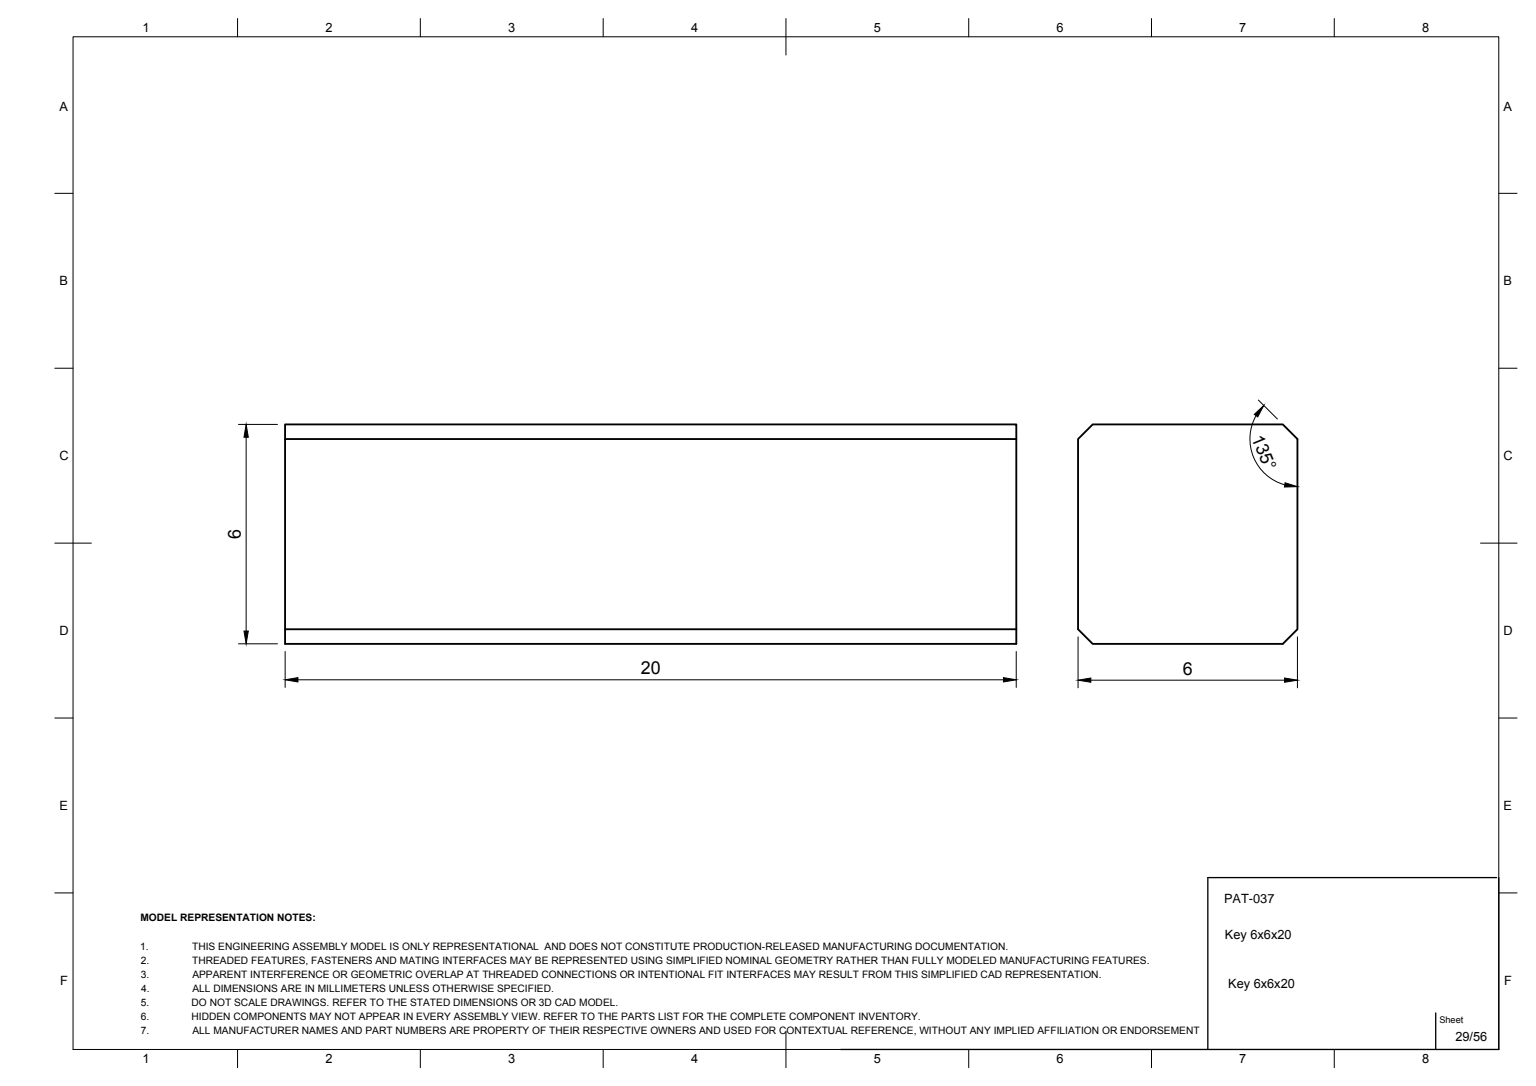
ISO-10303-21;
HEADER;
/* Generated by software containing ST-Developer
 * from STEP Tools, Inc. (www.steptools.com) 
 */

FILE_DESCRIPTION(
/* description */ ('Flywheel Crank-Slider'),
/* implementation_level */ '2;1');

FILE_NAME(
/* name */ 'Key 6x6x20.step',
/* time_stamp */ '2026-10-28T03:23:13-07:00',
/* author */ (''),
/* organization */ (''),
/* preprocessor_version */ 'ST-DEVELOPER v20.2',
/* originating_system */ 'Autodesk Translation Framework v15.17.0.0',
/* authorisation */ '');

FILE_SCHEMA (('AUTOMOTIVE_DESIGN { 1 0 10303 214 3 1 1 }'));
ENDSEC;

DATA;
#10=MECHANICAL_DESIGN_GEOMETRIC_PRESENTATION_REPRESENTATION('',(#699),#17322);
#594=SHAPE_REPRESENTATION_RELATIONSHIP('SRR','None',#17592,#646);
#646=ADVANCED_BREP_SHAPE_REPRESENTATION('',(#756),#17296);
#699=STYLED_ITEM('',(#17931),#756);
#756=MANIFOLD_SOLID_BREP('Body1',#9081);
#1211=PLANE('',#10312);
#1212=PLANE('',#10313);
#1213=PLANE('',#10314);
#1214=PLANE('',#10315);
#1215=PLANE('',#10316);
#1216=PLANE('',#10317);
#1217=PLANE('',#10318);
#1218=PLANE('',#10319);
#1219=PLANE('',#10320);
#1220=PLANE('',#10321);
#1656=FACE_OUTER_BOUND('',#2336,.T.);
#1657=FACE_OUTER_BOUND('',#2337,.T.);
#1658=FACE_OUTER_BOUND('',#2338,.T.);
#1659=FACE_OUTER_BOUND('',#2339,.T.);
#1660=FACE_OUTER_BOUND('',#2340,.T.);
#1661=FACE_OUTER_BOUND('',#2341,.T.);
#1662=FACE_OUTER_BOUND('',#2342,.T.);
#1663=FACE_OUTER_BOUND('',#2343,.T.);
#1664=FACE_OUTER_BOUND('',#2344,.T.);
#1665=FACE_OUTER_BOUND('',#2345,.T.);
#2336=EDGE_LOOP('',(#7516,#7517,#7518,#7519,#7520,#7521,#7522,#7523));
#2337=EDGE_LOOP('',(#7524,#7525,#7526,#7527));
#2338=EDGE_LOOP('',(#7528,#7529,#7530,#7531));
#2339=EDGE_LOOP('',(#7532,#7533,#7534,#7535));
#2340=EDGE_LOOP('',(#7536,#7537,#7538,#7539));
#2341=EDGE_LOOP('',(#7540,#7541,#7542,#7543,#7544,#7545,#7546,#7547));
#2342=EDGE_LOOP('',(#7548,#7549,#7550,#7551));
#2343=EDGE_LOOP('',(#7552,#7553,#7554,#7555));
#2344=EDGE_LOOP('',(#7556,#7557,#7558,#7559));
#2345=EDGE_LOOP('',(#7560,#7561,#7562,#7563));
#3023=LINE('',#15847,#3634);
#3024=LINE('',#15849,#3635);
#3025=LINE('',#15851,#3636);
#3026=LINE('',#15853,#3637);
#3027=LINE('',#15855,#3638);
#3028=LINE('',#15857,#3639);
#3029=LINE('',#15859,#3640);
#3030=LINE('',#15860,#3641);
#3031=LINE('',#15863,#3642);
#3032=LINE('',#15865,#3643);
#3033=LINE('',#15866,#3644);
#3034=LINE('',#15869,#3645);
#3035=LINE('',#15870,#3646);
#3036=LINE('',#15873,#3647);
#3037=LINE('',#15874,#3648);
#3038=LINE('',#15877,#3649);
#3039=LINE('',#15878,#3650);
#3040=LINE('',#15882,#3651);
#3041=LINE('',#15883,#3652);
#3042=LINE('',#15885,#3653);
#3043=LINE('',#15886,#3654);
#3044=LINE('',#15888,#3655);
#3045=LINE('',#15890,#3656);
#3046=LINE('',#15892,#3657);
#3634=VECTOR('',#12493,1.);
#3635=VECTOR('',#12494,1.);
#3636=VECTOR('',#12495,1.);
#3637=VECTOR('',#12496,1.);
#3638=VECTOR('',#12497,1.);
#3639=VECTOR('',#12498,1.);
#3640=VECTOR('',#12499,1.);
#3641=VECTOR('',#12500,1.);
#3642=VECTOR('',#12503,1.);
#3643=VECTOR('',#12504,1.);
#3644=VECTOR('',#12505,1.);
#3645=VECTOR('',#12508,1.);
#3646=VECTOR('',#12509,1.);
#3647=VECTOR('',#12512,1.);
#3648=VECTOR('',#12513,1.);
#3649=VECTOR('',#12516,1.);
#3650=VECTOR('',#12517,1.);
#3651=VECTOR('',#12520,1.);
#3652=VECTOR('',#12521,1.);
#3653=VECTOR('',#12522,1.);
#3654=VECTOR('',#12523,1.);
#3655=VECTOR('',#12526,1.);
#3656=VECTOR('',#12529,1.);
#3657=VECTOR('',#12532,1.);
#4739=VERTEX_POINT('',#15845);
#4740=VERTEX_POINT('',#15846);
#4741=VERTEX_POINT('',#15848);
#4742=VERTEX_POINT('',#15850);
#4743=VERTEX_POINT('',#15852);
#4744=VERTEX_POINT('',#15854);
#4745=VERTEX_POINT('',#15856);
#4746=VERTEX_POINT('',#15858);
#4747=VERTEX_POINT('',#15862);
#4748=VERTEX_POINT('',#15864);
#4749=VERTEX_POINT('',#15868);
#4750=VERTEX_POINT('',#15872);
#4751=VERTEX_POINT('',#15876);
#4752=VERTEX_POINT('',#15880);
#4753=VERTEX_POINT('',#15881);
#4754=VERTEX_POINT('',#15884);
#5715=EDGE_CURVE('',#4739,#4740,#3023,.T.);
#5716=EDGE_CURVE('',#4741,#4739,#3024,.T.);
#5717=EDGE_CURVE('',#4742,#4741,#3025,.T.);
#5718=EDGE_CURVE('',#4743,#4742,#3026,.T.);
#5719=EDGE_CURVE('',#4744,#4743,#3027,.T.);
#5720=EDGE_CURVE('',#4745,#4744,#3028,.T.);
#5721=EDGE_CURVE('',#4746,#4745,#3029,.T.);
#5722=EDGE_CURVE('',#4740,#4746,#3030,.T.);
#5723=EDGE_CURVE('',#4743,#4747,#3031,.T.);
#5724=EDGE_CURVE('',#4747,#4748,#3032,.T.);
#5725=EDGE_CURVE('',#4748,#4744,#3033,.T.);
#5726=EDGE_CURVE('',#4749,#4742,#3034,.T.);
#5727=EDGE_CURVE('',#4749,#4747,#3035,.T.);
#5728=EDGE_CURVE('',#4741,#4750,#3036,.T.);
#5729=EDGE_CURVE('',#4750,#4749,#3037,.T.);
#5730=EDGE_CURVE('',#4751,#4739,#3038,.T.);
#5731=EDGE_CURVE('',#4751,#4750,#3039,.T.);
#5732=EDGE_CURVE('',#4752,#4753,#3040,.T.);
#5733=EDGE_CURVE('',#4748,#4752,#3041,.T.);
#5734=EDGE_CURVE('',#4754,#4751,#3042,.T.);
#5735=EDGE_CURVE('',#4753,#4754,#3043,.T.);
#5736=EDGE_CURVE('',#4745,#4752,#3044,.T.);
#5737=EDGE_CURVE('',#4740,#4754,#3045,.T.);
#5738=EDGE_CURVE('',#4753,#4746,#3046,.T.);
#7516=ORIENTED_EDGE('',*,*,#5715,.F.);
#7517=ORIENTED_EDGE('',*,*,#5716,.F.);
#7518=ORIENTED_EDGE('',*,*,#5717,.F.);
#7519=ORIENTED_EDGE('',*,*,#5718,.F.);
#7520=ORIENTED_EDGE('',*,*,#5719,.F.);
#7521=ORIENTED_EDGE('',*,*,#5720,.F.);
#7522=ORIENTED_EDGE('',*,*,#5721,.F.);
#7523=ORIENTED_EDGE('',*,*,#5722,.F.);
#7524=ORIENTED_EDGE('',*,*,#5719,.T.);
#7525=ORIENTED_EDGE('',*,*,#5723,.T.);
#7526=ORIENTED_EDGE('',*,*,#5724,.T.);
#7527=ORIENTED_EDGE('',*,*,#5725,.T.);
#7528=ORIENTED_EDGE('',*,*,#5718,.T.);
#7529=ORIENTED_EDGE('',*,*,#5726,.F.);
#7530=ORIENTED_EDGE('',*,*,#5727,.T.);
#7531=ORIENTED_EDGE('',*,*,#5723,.F.);
#7532=ORIENTED_EDGE('',*,*,#5717,.T.);
#7533=ORIENTED_EDGE('',*,*,#5728,.T.);
#7534=ORIENTED_EDGE('',*,*,#5729,.T.);
#7535=ORIENTED_EDGE('',*,*,#5726,.T.);
#7536=ORIENTED_EDGE('',*,*,#5716,.T.);
#7537=ORIENTED_EDGE('',*,*,#5730,.F.);
#7538=ORIENTED_EDGE('',*,*,#5731,.T.);
#7539=ORIENTED_EDGE('',*,*,#5728,.F.);
#7540=ORIENTED_EDGE('',*,*,#5732,.F.);
#7541=ORIENTED_EDGE('',*,*,#5733,.F.);
#7542=ORIENTED_EDGE('',*,*,#5724,.F.);
#7543=ORIENTED_EDGE('',*,*,#5727,.F.);
#7544=ORIENTED_EDGE('',*,*,#5729,.F.);
#7545=ORIENTED_EDGE('',*,*,#5731,.F.);
#7546=ORIENTED_EDGE('',*,*,#5734,.F.);
#7547=ORIENTED_EDGE('',*,*,#5735,.F.);
#7548=ORIENTED_EDGE('',*,*,#5720,.T.);
#7549=ORIENTED_EDGE('',*,*,#5725,.F.);
#7550=ORIENTED_EDGE('',*,*,#5733,.T.);
#7551=ORIENTED_EDGE('',*,*,#5736,.F.);
#7552=ORIENTED_EDGE('',*,*,#5715,.T.);
#7553=ORIENTED_EDGE('',*,*,#5737,.T.);
#7554=ORIENTED_EDGE('',*,*,#5734,.T.);
#7555=ORIENTED_EDGE('',*,*,#5730,.T.);
#7556=ORIENTED_EDGE('',*,*,#5721,.T.);
#7557=ORIENTED_EDGE('',*,*,#5736,.T.);
#7558=ORIENTED_EDGE('',*,*,#5732,.T.);
#7559=ORIENTED_EDGE('',*,*,#5738,.T.);
#7560=ORIENTED_EDGE('',*,*,#5722,.T.);
#7561=ORIENTED_EDGE('',*,*,#5738,.F.);
#7562=ORIENTED_EDGE('',*,*,#5735,.T.);
#7563=ORIENTED_EDGE('',*,*,#5737,.F.);
#8847=ADVANCED_FACE('',(#1656),#1211,.F.);
#8848=ADVANCED_FACE('',(#1657),#1212,.T.);
#8849=ADVANCED_FACE('',(#1658),#1213,.T.);
#8850=ADVANCED_FACE('',(#1659),#1214,.T.);
#8851=ADVANCED_FACE('',(#1660),#1215,.T.);
#8852=ADVANCED_FACE('',(#1661),#1216,.T.);
#8853=ADVANCED_FACE('',(#1662),#1217,.F.);
#8854=ADVANCED_FACE('',(#1663),#1218,.T.);
#8855=ADVANCED_FACE('',(#1664),#1219,.T.);
#8856=ADVANCED_FACE('',(#1665),#1220,.T.);
#9081=CLOSED_SHELL('',(#8847,#8848,#8849,#8850,#8851,#8852,#8853,#8854,
#8855,#8856));
#10311=AXIS2_PLACEMENT_3D('',#15843,#12489,#12490);
#10312=AXIS2_PLACEMENT_3D('',#15844,#12491,#12492);
#10313=AXIS2_PLACEMENT_3D('',#15861,#12501,#12502);
#10314=AXIS2_PLACEMENT_3D('',#15867,#12506,#12507);
#10315=AXIS2_PLACEMENT_3D('',#15871,#12510,#12511);
#10316=AXIS2_PLACEMENT_3D('',#15875,#12514,#12515);
#10317=AXIS2_PLACEMENT_3D('',#15879,#12518,#12519);
#10318=AXIS2_PLACEMENT_3D('',#15887,#12524,#12525);
#10319=AXIS2_PLACEMENT_3D('',#15889,#12527,#12528);
#10320=AXIS2_PLACEMENT_3D('',#15891,#12530,#12531);
#10321=AXIS2_PLACEMENT_3D('',#15893,#12533,#12534);
#12489=DIRECTION('axis',(0.,0.,1.));
#12490=DIRECTION('refdir',(1.,0.,0.));
#12491=DIRECTION('center_axis',(1.,0.,0.));
#12492=DIRECTION('ref_axis',(0.,0.,-1.));
#12493=DIRECTION('',(0.,-0.707106781186547,-0.707106781186548));
#12494=DIRECTION('',(0.,-1.,0.));
#12495=DIRECTION('',(0.,-0.707106781186547,0.707106781186548));
#12496=DIRECTION('',(0.,0.,1.));
#12497=DIRECTION('',(0.,0.707106781186547,0.707106781186548));
#12498=DIRECTION('',(0.,1.,0.));
#12499=DIRECTION('',(0.,0.707106781186547,-0.707106781186548));
#12500=DIRECTION('',(0.,0.,-1.));
#12501=DIRECTION('center_axis',(0.,0.707106781186548,-0.707106781186547));
#12502=DIRECTION('ref_axis',(-1.,0.,0.));
#12503=DIRECTION('',(1.,0.,0.));
#12504=DIRECTION('',(0.,-0.707106781186547,-0.707106781186548));
#12505=DIRECTION('',(-1.,0.,0.));
#12506=DIRECTION('center_axis',(0.,1.,0.));
#12507=DIRECTION('ref_axis',(-1.,0.,0.));
#12508=DIRECTION('',(-1.,0.,0.));
#12509=DIRECTION('',(0.,0.,-1.));
#12510=DIRECTION('center_axis',(0.,0.707106781186548,0.707106781186547));
#12511=DIRECTION('ref_axis',(1.,0.,0.));
#12512=DIRECTION('',(1.,0.,0.));
#12513=DIRECTION('',(0.,0.707106781186547,-0.707106781186548));
#12514=DIRECTION('center_axis',(0.,0.,1.));
#12515=DIRECTION('ref_axis',(1.,0.,0.));
#12516=DIRECTION('',(-1.,0.,0.));
#12517=DIRECTION('',(0.,1.,0.));
#12518=DIRECTION('center_axis',(1.,0.,0.));
#12519=DIRECTION('ref_axis',(0.,0.,-1.));
#12520=DIRECTION('',(0.,-0.707106781186547,0.707106781186548));
#12521=DIRECTION('',(0.,-1.,0.));
#12522=DIRECTION('',(0.,0.707106781186547,0.707106781186548));
#12523=DIRECTION('',(0.,0.,1.));
#12524=DIRECTION('center_axis',(0.,0.,1.));
#12525=DIRECTION('ref_axis',(1.,0.,0.));
#12526=DIRECTION('',(1.,0.,0.));
#12527=DIRECTION('center_axis',(0.,-0.707106781186548,0.707106781186547));
#12528=DIRECTION('ref_axis',(1.,0.,0.));
#12529=DIRECTION('',(1.,0.,0.));
#12530=DIRECTION('center_axis',(0.,-0.707106781186548,-0.707106781186547));
#12531=DIRECTION('ref_axis',(-1.,0.,0.));
#12532=DIRECTION('',(-1.,0.,0.));
#12533=DIRECTION('center_axis',(0.,-1.,0.));
#12534=DIRECTION('ref_axis',(1.,0.,0.));
#15843=CARTESIAN_POINT('',(0.,0.,0.));
#15844=CARTESIAN_POINT('Origin',(-1.,0.,0.35));
#15845=CARTESIAN_POINT('',(-1.,-0.26,0.6));
#15846=CARTESIAN_POINT('',(-1.,-0.3,0.56));
#15847=CARTESIAN_POINT('',(-1.,-0.2675,0.5925));
#15848=CARTESIAN_POINT('',(-1.,0.26,0.6));
#15849=CARTESIAN_POINT('',(-1.,0.,0.6));
#15850=CARTESIAN_POINT('',(-1.,0.3,0.56));
#15851=CARTESIAN_POINT('',(-1.,0.2675,0.5925));
#15852=CARTESIAN_POINT('',(-1.,0.3,0.04));
#15853=CARTESIAN_POINT('',(-1.,0.3,0.175));
#15854=CARTESIAN_POINT('',(-1.,0.26,0.));
#15855=CARTESIAN_POINT('',(-1.,0.2925,0.0325));
#15856=CARTESIAN_POINT('',(-1.,-0.26,0.));
#15857=CARTESIAN_POINT('',(-1.,0.,0.));
#15858=CARTESIAN_POINT('',(-1.,-0.3,0.04));
#15859=CARTESIAN_POINT('',(-1.,-0.2925,0.0325));
#15860=CARTESIAN_POINT('',(-1.,-0.3,0.175));
#15861=CARTESIAN_POINT('Origin',(0.75,0.28,0.02));
#15862=CARTESIAN_POINT('',(1.,0.3,0.04));
#15863=CARTESIAN_POINT('',(0.75,0.3,0.04));
#15864=CARTESIAN_POINT('',(1.,0.26,0.));
#15865=CARTESIAN_POINT('',(1.,0.2925,0.0325));
#15866=CARTESIAN_POINT('',(0.75,0.26,0.));
#15867=CARTESIAN_POINT('Origin',(1.5,0.3,0.));
#15868=CARTESIAN_POINT('',(1.,0.3,0.56));
#15869=CARTESIAN_POINT('',(0.75,0.3,0.56));
#15870=CARTESIAN_POINT('',(1.,0.3,0.175));
#15871=CARTESIAN_POINT('Origin',(0.75,0.28,0.58));
#15872=CARTESIAN_POINT('',(1.,0.26,0.6));
#15873=CARTESIAN_POINT('',(0.75,0.26,0.6));
#15874=CARTESIAN_POINT('',(1.,0.2675,0.5925));
#15875=CARTESIAN_POINT('Origin',(0.,0.,0.6));
#15876=CARTESIAN_POINT('',(1.,-0.26,0.6));
#15877=CARTESIAN_POINT('',(-0.75,-0.26,0.6));
#15878=CARTESIAN_POINT('',(1.,0.,0.6));
#15879=CARTESIAN_POINT('Origin',(1.,0.,0.35));
#15880=CARTESIAN_POINT('',(1.,-0.26,0.));
#15881=CARTESIAN_POINT('',(1.,-0.3,0.04));
#15882=CARTESIAN_POINT('',(1.,-0.2925,0.0325));
#15883=CARTESIAN_POINT('',(1.,0.,0.));
#15884=CARTESIAN_POINT('',(1.,-0.3,0.56));
#15885=CARTESIAN_POINT('',(1.,-0.2675,0.5925));
#15886=CARTESIAN_POINT('',(1.,-0.3,0.175));
#15887=CARTESIAN_POINT('Origin',(0.,0.,0.));
#15888=CARTESIAN_POINT('',(-0.75,-0.26,0.));
#15889=CARTESIAN_POINT('Origin',(-0.75,-0.28,0.58));
#15890=CARTESIAN_POINT('',(-0.75,-0.3,0.56));
#15891=CARTESIAN_POINT('Origin',(-0.75,-0.28,0.02));
#15892=CARTESIAN_POINT('',(-0.75,-0.3,0.04));
#15893=CARTESIAN_POINT('Origin',(-1.5,-0.3,0.));
#17235=UNCERTAINTY_MEASURE_WITH_UNIT(LENGTH_MEASURE(0.001),#17323,
'DISTANCE_ACCURACY_VALUE',
'Maximum model space distance between geometric entities at asserted c
onnectivities');
#17261=UNCERTAINTY_MEASURE_WITH_UNIT(LENGTH_MEASURE(0.001),#17323,
'DISTANCE_ACCURACY_VALUE',
'Maximum model space distance between geometric entities at asserted c
onnectivities');
#17296=(
GEOMETRIC_REPRESENTATION_CONTEXT(3)
GLOBAL_UNCERTAINTY_ASSIGNED_CONTEXT((#17235))
GLOBAL_UNIT_ASSIGNED_CONTEXT((#17323,#17325,#17326))
REPRESENTATION_CONTEXT('','3D')
);
#17322=(
GEOMETRIC_REPRESENTATION_CONTEXT(3)
GLOBAL_UNCERTAINTY_ASSIGNED_CONTEXT((#17261))
GLOBAL_UNIT_ASSIGNED_CONTEXT((#17323,#17325,#17326))
REPRESENTATION_CONTEXT('','3D')
);
#17323=(
LENGTH_UNIT()
NAMED_UNIT(*)
SI_UNIT(.CENTI.,.METRE.)
);
#17325=(
NAMED_UNIT(*)
PLANE_ANGLE_UNIT()
SI_UNIT($,.RADIAN.)
);
#17326=(
NAMED_UNIT(*)
SI_UNIT($,.STERADIAN.)
SOLID_ANGLE_UNIT()
);
#17361=SHAPE_DEFINITION_REPRESENTATION(#17423,#17592);
#17423=PRODUCT_DEFINITION_SHAPE('',$,#17653);
#17592=SHAPE_REPRESENTATION('',(#10311),#17296);
#17618=PRODUCT_DEFINITION_CONTEXT('part definition',#17800,'design');
#17653=PRODUCT_DEFINITION('Key 6x6x20','Key 6x6x20',#17713,#17618);
#17713=PRODUCT_DEFINITION_FORMATION('',$,#17836);
#17800=APPLICATION_CONTEXT(
'Core Data for Automotive Mechanical Design Process');
#17801=PRODUCT_CONTEXT('part definition',#17800,'mechanical');
#17836=PRODUCT('Key 6x6x20','Key 6x6x20','Key 6x6x20',(#17801));
#17925=COLOUR_RGB('Grey',0.48,0.52,0.57);
#17926=FILL_AREA_STYLE_COLOUR('',#17925);
#17927=FILL_AREA_STYLE('',(#17926));
#17928=SURFACE_STYLE_FILL_AREA(#17927);
#17929=SURFACE_SIDE_STYLE('',(#17928));
#17930=SURFACE_STYLE_USAGE(.BOTH.,#17929);
#17931=PRESENTATION_STYLE_ASSIGNMENT((#17930));
ENDSEC;
END-ISO-10303-21;
